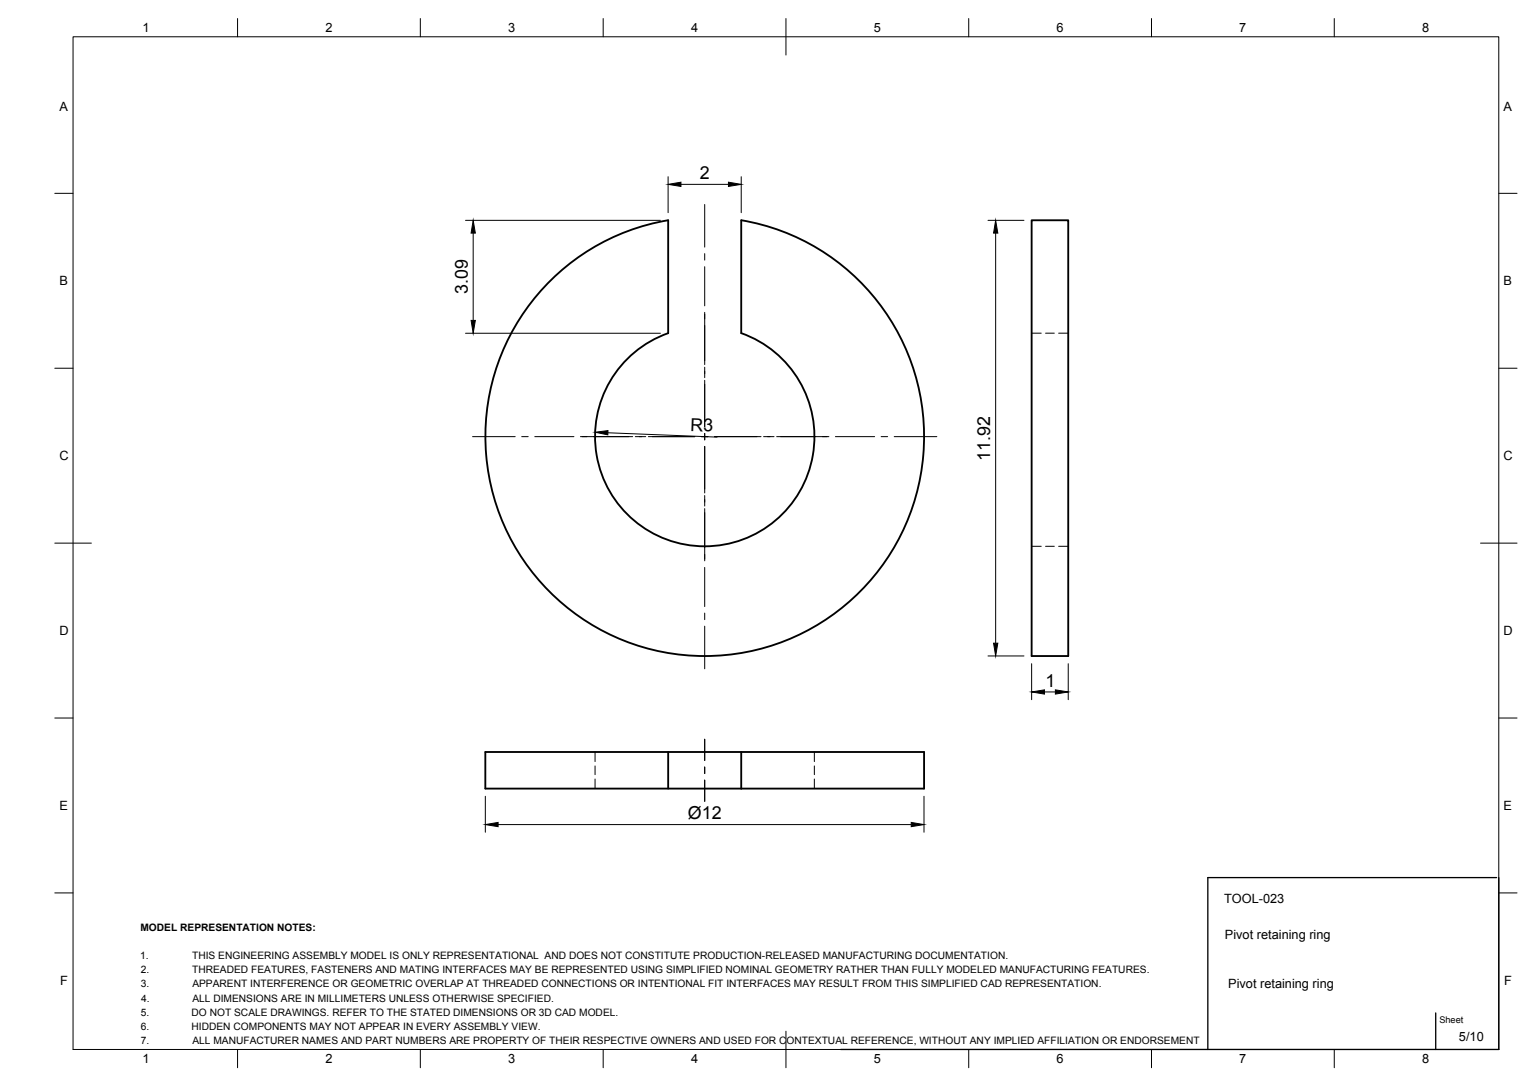
ISO-10303-21;
HEADER;
/* Generated by software containing ST-Developer
 * from STEP Tools, Inc. (www.steptools.com) 
 */

FILE_DESCRIPTION(
/* description */ (''),
/* implementation_level */ '2;1');

FILE_NAME(
/* name */ 'Pivot retaining ring.step',
/* time_stamp */ '2026-11-10T05:40:20-08:00',
/* author */ (''),
/* organization */ (''),
/* preprocessor_version */ 'ST-DEVELOPER v20.2',
/* originating_system */ 'Autodesk Translation Framework v15.17.0.0',
/* authorisation */ '');

FILE_SCHEMA (('AUTOMOTIVE_DESIGN { 1 0 10303 214 3 1 1 }'));
ENDSEC;

DATA;
#10=MECHANICAL_DESIGN_GEOMETRIC_PRESENTATION_REPRESENTATION('',(#574),#18580);
#556=SHAPE_REPRESENTATION_RELATIONSHIP('SRR','None',#18626,#565);
#565=ADVANCED_BREP_SHAPE_REPRESENTATION('',(#583),#18572);
#574=STYLED_ITEM('',(#18685),#583);
#583=MANIFOLD_SOLID_BREP('Body1',#6546);
#678=PLANE('',#6711);
#679=PLANE('',#6712);
#680=PLANE('',#6713);
#681=PLANE('',#6720);
#832=FACE_OUTER_BOUND('',#1217,.T.);
#833=FACE_OUTER_BOUND('',#1218,.T.);
#834=FACE_OUTER_BOUND('',#1219,.T.);
#835=FACE_OUTER_BOUND('',#1220,.T.);
#836=FACE_OUTER_BOUND('',#1221,.T.);
#837=FACE_OUTER_BOUND('',#1222,.T.);
#1217=EDGE_LOOP('',(#4310,#4311,#4312,#4313));
#1218=EDGE_LOOP('',(#4314,#4315,#4316,#4317));
#1219=EDGE_LOOP('',(#4318,#4319,#4320,#4321));
#1220=EDGE_LOOP('',(#4322,#4323,#4324,#4325));
#1221=EDGE_LOOP('',(#4326,#4327,#4328,#4329));
#1222=EDGE_LOOP('',(#4330,#4331,#4332,#4333));
#1676=LINE('',#8687,#2083);
#1677=LINE('',#8689,#2084);
#1678=LINE('',#8691,#2085);
#1679=LINE('',#8692,#2086);
#1680=LINE('',#8696,#2087);
#1681=LINE('',#8698,#2088);
#1682=LINE('',#8700,#2089);
#1683=LINE('',#8701,#2090);
#2083=VECTOR('',#7319,1.);
#2084=VECTOR('',#7320,1.);
#2085=VECTOR('',#7321,1.);
#2086=VECTOR('',#7322,1.);
#2087=VECTOR('',#7325,1.);
#2088=VECTOR('',#7326,1.);
#2089=VECTOR('',#7327,1.);
#2090=VECTOR('',#7328,1.);
#2441=CIRCLE('',#6714,0.6);
#2442=CIRCLE('',#6715,0.3);
#2443=CIRCLE('',#6717,0.3);
#2444=CIRCLE('',#6719,0.6);
#2637=VERTEX_POINT('',#8685);
#2638=VERTEX_POINT('',#8686);
#2639=VERTEX_POINT('',#8688);
#2640=VERTEX_POINT('',#8690);
#2641=VERTEX_POINT('',#8694);
#2642=VERTEX_POINT('',#8695);
#2643=VERTEX_POINT('',#8697);
#2644=VERTEX_POINT('',#8699);
#3278=EDGE_CURVE('',#2637,#2638,#1676,.T.);
#3279=EDGE_CURVE('',#2639,#2637,#1677,.T.);
#3280=EDGE_CURVE('',#2640,#2639,#1678,.T.);
#3281=EDGE_CURVE('',#2638,#2640,#1679,.T.);
#3282=EDGE_CURVE('',#2641,#2642,#1680,.T.);
#3283=EDGE_CURVE('',#2643,#2641,#1681,.T.);
#3284=EDGE_CURVE('',#2644,#2643,#1682,.T.);
#3285=EDGE_CURVE('',#2642,#2644,#1683,.T.);
#3286=EDGE_CURVE('',#2639,#2644,#2441,.T.);
#3287=EDGE_CURVE('',#2642,#2637,#2442,.T.);
#3288=EDGE_CURVE('',#2641,#2638,#2443,.T.);
#3289=EDGE_CURVE('',#2640,#2643,#2444,.T.);
#4310=ORIENTED_EDGE('',*,*,#3278,.F.);
#4311=ORIENTED_EDGE('',*,*,#3279,.F.);
#4312=ORIENTED_EDGE('',*,*,#3280,.F.);
#4313=ORIENTED_EDGE('',*,*,#3281,.F.);
#4314=ORIENTED_EDGE('',*,*,#3282,.F.);
#4315=ORIENTED_EDGE('',*,*,#3283,.F.);
#4316=ORIENTED_EDGE('',*,*,#3284,.F.);
#4317=ORIENTED_EDGE('',*,*,#3285,.F.);
#4318=ORIENTED_EDGE('',*,*,#3285,.T.);
#4319=ORIENTED_EDGE('',*,*,#3286,.F.);
#4320=ORIENTED_EDGE('',*,*,#3279,.T.);
#4321=ORIENTED_EDGE('',*,*,#3287,.F.);
#4322=ORIENTED_EDGE('',*,*,#3282,.T.);
#4323=ORIENTED_EDGE('',*,*,#3287,.T.);
#4324=ORIENTED_EDGE('',*,*,#3278,.T.);
#4325=ORIENTED_EDGE('',*,*,#3288,.F.);
#4326=ORIENTED_EDGE('',*,*,#3284,.T.);
#4327=ORIENTED_EDGE('',*,*,#3289,.F.);
#4328=ORIENTED_EDGE('',*,*,#3280,.T.);
#4329=ORIENTED_EDGE('',*,*,#3286,.T.);
#4330=ORIENTED_EDGE('',*,*,#3283,.T.);
#4331=ORIENTED_EDGE('',*,*,#3288,.T.);
#4332=ORIENTED_EDGE('',*,*,#3281,.T.);
#4333=ORIENTED_EDGE('',*,*,#3289,.T.);
#6043=CYLINDRICAL_SURFACE('',#6716,0.3);
#6044=CYLINDRICAL_SURFACE('',#6718,0.6);
#6204=ADVANCED_FACE('',(#832),#678,.F.);
#6205=ADVANCED_FACE('',(#833),#679,.F.);
#6206=ADVANCED_FACE('',(#834),#680,.F.);
#6207=ADVANCED_FACE('',(#835),#6043,.F.);
#6208=ADVANCED_FACE('',(#836),#6044,.T.);
#6209=ADVANCED_FACE('',(#837),#681,.T.);
#6546=CLOSED_SHELL('',(#6204,#6205,#6206,#6207,#6208,#6209));
#6710=AXIS2_PLACEMENT_3D('',#8683,#7315,#7316);
#6711=AXIS2_PLACEMENT_3D('',#8684,#7317,#7318);
#6712=AXIS2_PLACEMENT_3D('',#8693,#7323,#7324);
#6713=AXIS2_PLACEMENT_3D('',#8702,#7329,#7330);
#6714=AXIS2_PLACEMENT_3D('',#8703,#7331,#7332);
#6715=AXIS2_PLACEMENT_3D('',#8704,#7333,#7334);
#6716=AXIS2_PLACEMENT_3D('',#8705,#7335,#7336);
#6717=AXIS2_PLACEMENT_3D('',#8706,#7337,#7338);
#6718=AXIS2_PLACEMENT_3D('',#8707,#7339,#7340);
#6719=AXIS2_PLACEMENT_3D('',#8708,#7341,#7342);
#6720=AXIS2_PLACEMENT_3D('',#8709,#7343,#7344);
#7315=DIRECTION('axis',(0.,0.,1.));
#7316=DIRECTION('refdir',(1.,0.,0.));
#7317=DIRECTION('center_axis',(-1.,0.,0.));
#7318=DIRECTION('ref_axis',(0.,1.,0.));
#7319=DIRECTION('',(0.,0.,1.));
#7320=DIRECTION('',(0.,-1.,0.));
#7321=DIRECTION('',(0.,0.,-1.));
#7322=DIRECTION('',(0.,1.,0.));
#7323=DIRECTION('center_axis',(1.,0.,0.));
#7324=DIRECTION('ref_axis',(0.,-1.,0.));
#7325=DIRECTION('',(0.,0.,-1.));
#7326=DIRECTION('',(0.,-1.,0.));
#7327=DIRECTION('',(0.,0.,1.));
#7328=DIRECTION('',(0.,1.,0.));
#7329=DIRECTION('center_axis',(0.,0.,1.));
#7330=DIRECTION('ref_axis',(1.,0.,0.));
#7331=DIRECTION('center_axis',(0.,0.,1.));
#7332=DIRECTION('ref_axis',(1.,0.,0.));
#7333=DIRECTION('center_axis',(0.,0.,-1.));
#7334=DIRECTION('ref_axis',(1.,0.,0.));
#7335=DIRECTION('center_axis',(0.,0.,1.));
#7336=DIRECTION('ref_axis',(6.12323399573677E-17,-1.,0.));
#7337=DIRECTION('center_axis',(0.,0.,-1.));
#7338=DIRECTION('ref_axis',(1.,0.,0.));
#7339=DIRECTION('center_axis',(0.,0.,1.));
#7340=DIRECTION('ref_axis',(6.12323399573677E-17,-1.,0.));
#7341=DIRECTION('center_axis',(0.,0.,1.));
#7342=DIRECTION('ref_axis',(1.,0.,0.));
#7343=DIRECTION('center_axis',(0.,0.,1.));
#7344=DIRECTION('ref_axis',(1.,0.,0.));
#8683=CARTESIAN_POINT('',(0.,0.,0.));
#8684=CARTESIAN_POINT('Origin',(-0.1,0.,0.1));
#8685=CARTESIAN_POINT('',(-0.1,0.282842712474619,0.));
#8686=CARTESIAN_POINT('',(-0.1,0.282842712474619,0.1));
#8687=CARTESIAN_POINT('',(-0.1,0.282842712474619,0.));
#8688=CARTESIAN_POINT('',(-0.1,0.591607978309962,0.));
#8689=CARTESIAN_POINT('',(-0.1,0.,0.));
#8690=CARTESIAN_POINT('',(-0.1,0.591607978309962,0.1));
#8691=CARTESIAN_POINT('',(-0.1,0.591607978309962,0.));
#8692=CARTESIAN_POINT('',(-0.1,0.,0.1));
#8693=CARTESIAN_POINT('Origin',(0.1,1.2,0.1));
#8694=CARTESIAN_POINT('',(0.1,0.282842712474619,0.1));
#8695=CARTESIAN_POINT('',(0.1,0.282842712474619,0.));
#8696=CARTESIAN_POINT('',(0.1,0.282842712474619,0.));
#8697=CARTESIAN_POINT('',(0.1,0.591607978309962,0.1));
#8698=CARTESIAN_POINT('',(0.1,0.6,0.1));
#8699=CARTESIAN_POINT('',(0.1,0.591607978309962,0.));
#8700=CARTESIAN_POINT('',(0.1,0.591607978309962,0.));
#8701=CARTESIAN_POINT('',(0.1,0.6,0.));
#8702=CARTESIAN_POINT('Origin',(0.,0.,0.));
#8703=CARTESIAN_POINT('Origin',(0.,0.,0.));
#8704=CARTESIAN_POINT('Origin',(0.,0.,0.));
#8705=CARTESIAN_POINT('Origin',(0.,0.,0.));
#8706=CARTESIAN_POINT('Origin',(0.,0.,0.1));
#8707=CARTESIAN_POINT('Origin',(0.,0.,0.));
#8708=CARTESIAN_POINT('Origin',(0.,0.,0.1));
#8709=CARTESIAN_POINT('Origin',(0.,0.,0.1));
#18560=UNCERTAINTY_MEASURE_WITH_UNIT(LENGTH_MEASURE(0.001),#18581,
'DISTANCE_ACCURACY_VALUE',
'Maximum model space distance between geometric entities at asserted c
onnectivities');
#18568=UNCERTAINTY_MEASURE_WITH_UNIT(LENGTH_MEASURE(0.001),#18581,
'DISTANCE_ACCURACY_VALUE',
'Maximum model space distance between geometric entities at asserted c
onnectivities');
#18572=(
GEOMETRIC_REPRESENTATION_CONTEXT(3)
GLOBAL_UNCERTAINTY_ASSIGNED_CONTEXT((#18560))
GLOBAL_UNIT_ASSIGNED_CONTEXT((#18581,#18583,#18584))
REPRESENTATION_CONTEXT('','3D')
);
#18580=(
GEOMETRIC_REPRESENTATION_CONTEXT(3)
GLOBAL_UNCERTAINTY_ASSIGNED_CONTEXT((#18568))
GLOBAL_UNIT_ASSIGNED_CONTEXT((#18581,#18583,#18584))
REPRESENTATION_CONTEXT('','3D')
);
#18581=(
LENGTH_UNIT()
NAMED_UNIT(*)
SI_UNIT(.CENTI.,.METRE.)
);
#18583=(
NAMED_UNIT(*)
PLANE_ANGLE_UNIT()
SI_UNIT($,.RADIAN.)
);
#18584=(
NAMED_UNIT(*)
SI_UNIT($,.STERADIAN.)
SOLID_ANGLE_UNIT()
);
#18588=SHAPE_DEFINITION_REPRESENTATION(#18599,#18626);
#18599=PRODUCT_DEFINITION_SHAPE('',$,#18638);
#18626=SHAPE_REPRESENTATION('',(#6710),#18572);
#18634=PRODUCT_DEFINITION_CONTEXT('part definition',#18669,'design');
#18638=PRODUCT_DEFINITION('Pivot retaining ring','Pivot retaining ring',
#18649,#18634);
#18649=PRODUCT_DEFINITION_FORMATION('',$,#18674);
#18669=APPLICATION_CONTEXT(
'Core Data for Automotive Mechanical Design Process');
#18670=PRODUCT_CONTEXT('part definition',#18669,'mechanical');
#18674=PRODUCT('Pivot retaining ring','Pivot retaining ring',$,(#18670));
#18685=PRESENTATION_STYLE_ASSIGNMENT((#18693));
#18693=SURFACE_STYLE_USAGE(.BOTH.,#18701);
#18701=SURFACE_SIDE_STYLE('',(#18709));
#18709=SURFACE_STYLE_FILL_AREA(#18717);
#18717=FILL_AREA_STYLE('Dark gray',(#18725));
#18725=FILL_AREA_STYLE_COLOUR('Dark gray',#18733);
#18733=COLOUR_RGB('Dark gray',0.250980392156863,0.282352941176471,0.32156862745098);
ENDSEC;
END-ISO-10303-21;
